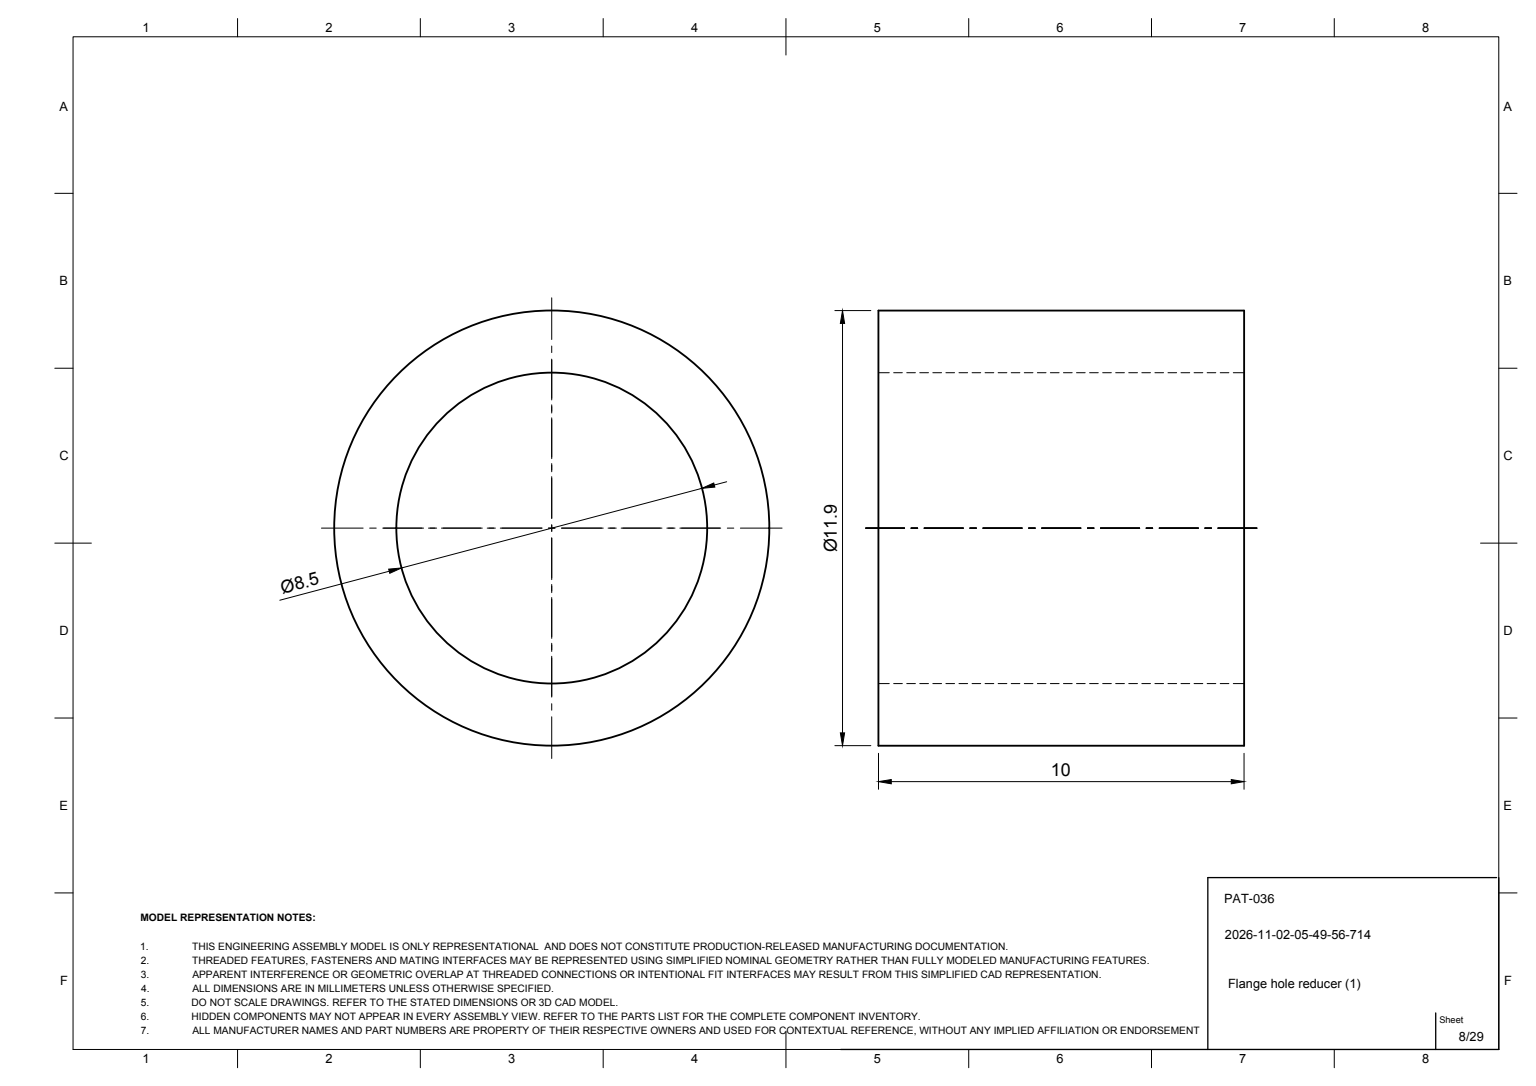
ISO-10303-21;
HEADER;
/* Generated by software containing ST-Developer
 * from STEP Tools, Inc. (www.steptools.com) 
 */

FILE_DESCRIPTION(
/* description */ ('Flange-mounted spindle'),
/* implementation_level */ '2;1');

FILE_NAME(
/* name */ 'Flange hole reducer (1).step',
/* time_stamp */ '2026-10-27T10:49:51-07:00',
/* author */ (''),
/* organization */ (''),
/* preprocessor_version */ 'ST-DEVELOPER v20.2',
/* originating_system */ 'Autodesk Translation Framework v15.17.0.0',
/* authorisation */ '');

FILE_SCHEMA (('AUTOMOTIVE_DESIGN { 1 0 10303 214 3 1 1 }'));
ENDSEC;

DATA;
#10=MECHANICAL_DESIGN_GEOMETRIC_PRESENTATION_REPRESENTATION('',(#341),#11764);
#287=SHAPE_REPRESENTATION_RELATIONSHIP('SRR','None',#11883,#314);
#314=ADVANCED_BREP_SHAPE_REPRESENTATION('',(#369),#11738);
#341=STYLED_ITEM('',(#12113),#369);
#369=MANIFOLD_SOLID_BREP('Body1',#6133);
#411=FACE_BOUND('',#1069,.T.);
#412=FACE_BOUND('',#1071,.T.);
#522=PLANE('',#6520);
#523=PLANE('',#6521);
#701=FACE_OUTER_BOUND('',#1066,.T.);
#702=FACE_OUTER_BOUND('',#1067,.T.);
#703=FACE_OUTER_BOUND('',#1068,.T.);
#704=FACE_OUTER_BOUND('',#1070,.T.);
#1066=EDGE_LOOP('',(#4131,#4132,#4133,#4134));
#1067=EDGE_LOOP('',(#4135,#4136,#4137,#4138));
#1068=EDGE_LOOP('',(#4139));
#1069=EDGE_LOOP('',(#4140));
#1070=EDGE_LOOP('',(#4141));
#1071=EDGE_LOOP('',(#4142));
#1520=LINE('',#9270,#1942);
#1521=LINE('',#9276,#1943);
#1942=VECTOR('',#7363,0.425);
#1943=VECTOR('',#7370,0.595);
#2345=CIRCLE('',#6515,0.425);
#2346=CIRCLE('',#6516,0.425);
#2347=CIRCLE('',#6518,0.595);
#2348=CIRCLE('',#6519,0.595);
#2691=VERTEX_POINT('',#9267);
#2692=VERTEX_POINT('',#9269);
#2693=VERTEX_POINT('',#9273);
#2694=VERTEX_POINT('',#9275);
#3258=EDGE_CURVE('',#2691,#2691,#2345,.T.);
#3259=EDGE_CURVE('',#2691,#2692,#1520,.T.);
#3260=EDGE_CURVE('',#2692,#2692,#2346,.T.);
#3261=EDGE_CURVE('',#2693,#2693,#2347,.T.);
#3262=EDGE_CURVE('',#2693,#2694,#1521,.T.);
#3263=EDGE_CURVE('',#2694,#2694,#2348,.T.);
#4131=ORIENTED_EDGE('',*,*,#3258,.F.);
#4132=ORIENTED_EDGE('',*,*,#3259,.T.);
#4133=ORIENTED_EDGE('',*,*,#3260,.T.);
#4134=ORIENTED_EDGE('',*,*,#3259,.F.);
#4135=ORIENTED_EDGE('',*,*,#3261,.F.);
#4136=ORIENTED_EDGE('',*,*,#3262,.T.);
#4137=ORIENTED_EDGE('',*,*,#3263,.T.);
#4138=ORIENTED_EDGE('',*,*,#3262,.F.);
#4139=ORIENTED_EDGE('',*,*,#3261,.T.);
#4140=ORIENTED_EDGE('',*,*,#3258,.T.);
#4141=ORIENTED_EDGE('',*,*,#3263,.F.);
#4142=ORIENTED_EDGE('',*,*,#3260,.F.);
#5636=CYLINDRICAL_SURFACE('',#6514,0.425);
#5637=CYLINDRICAL_SURFACE('',#6517,0.595);
#5812=ADVANCED_FACE('',(#701),#5636,.F.);
#5813=ADVANCED_FACE('',(#702),#5637,.T.);
#5814=ADVANCED_FACE('',(#703,#411),#522,.T.);
#5815=ADVANCED_FACE('',(#704,#412),#523,.F.);
#6133=CLOSED_SHELL('',(#5812,#5813,#5814,#5815));
#6513=AXIS2_PLACEMENT_3D('',#9265,#7357,#7358);
#6514=AXIS2_PLACEMENT_3D('',#9266,#7359,#7360);
#6515=AXIS2_PLACEMENT_3D('',#9268,#7361,#7362);
#6516=AXIS2_PLACEMENT_3D('',#9271,#7364,#7365);
#6517=AXIS2_PLACEMENT_3D('',#9272,#7366,#7367);
#6518=AXIS2_PLACEMENT_3D('',#9274,#7368,#7369);
#6519=AXIS2_PLACEMENT_3D('',#9277,#7371,#7372);
#6520=AXIS2_PLACEMENT_3D('',#9278,#7373,#7374);
#6521=AXIS2_PLACEMENT_3D('',#9279,#7375,#7376);
#7357=DIRECTION('axis',(0.,0.,1.));
#7358=DIRECTION('refdir',(1.,0.,0.));
#7359=DIRECTION('center_axis',(0.,1.,0.));
#7360=DIRECTION('ref_axis',(1.,0.,0.));
#7361=DIRECTION('center_axis',(0.,-1.,0.));
#7362=DIRECTION('ref_axis',(1.,0.,0.));
#7363=DIRECTION('',(0.,-1.,0.));
#7364=DIRECTION('center_axis',(0.,-1.,0.));
#7365=DIRECTION('ref_axis',(1.,0.,0.));
#7366=DIRECTION('center_axis',(0.,1.,0.));
#7367=DIRECTION('ref_axis',(1.,0.,0.));
#7368=DIRECTION('center_axis',(0.,1.,0.));
#7369=DIRECTION('ref_axis',(1.,0.,0.));
#7370=DIRECTION('',(0.,-1.,0.));
#7371=DIRECTION('center_axis',(0.,1.,0.));
#7372=DIRECTION('ref_axis',(1.,0.,0.));
#7373=DIRECTION('center_axis',(0.,1.,0.));
#7374=DIRECTION('ref_axis',(1.,0.,0.));
#7375=DIRECTION('center_axis',(0.,1.,0.));
#7376=DIRECTION('ref_axis',(1.,0.,0.));
#9265=CARTESIAN_POINT('',(0.,0.,0.));
#9266=CARTESIAN_POINT('Origin',(-3.2,-0.5,11.2));
#9267=CARTESIAN_POINT('',(-3.625,0.5,11.2));
#9268=CARTESIAN_POINT('Origin',(-3.2,0.5,11.2));
#9269=CARTESIAN_POINT('',(-3.625,-0.5,11.2));
#9270=CARTESIAN_POINT('',(-3.625,-0.5,11.2));
#9271=CARTESIAN_POINT('Origin',(-3.2,-0.5,11.2));
#9272=CARTESIAN_POINT('Origin',(-3.2,-0.5,11.2));
#9273=CARTESIAN_POINT('',(-3.795,0.5,11.2));
#9274=CARTESIAN_POINT('Origin',(-3.2,0.5,11.2));
#9275=CARTESIAN_POINT('',(-3.795,-0.5,11.2));
#9276=CARTESIAN_POINT('',(-3.795,-0.5,11.2));
#9277=CARTESIAN_POINT('Origin',(-3.2,-0.5,11.2));
#9278=CARTESIAN_POINT('Origin',(-3.2,0.5,11.2));
#9279=CARTESIAN_POINT('Origin',(-3.2,-0.5,11.2));
#11706=UNCERTAINTY_MEASURE_WITH_UNIT(LENGTH_MEASURE(0.001),#11765,
'DISTANCE_ACCURACY_VALUE',
'Maximum model space distance between geometric entities at asserted c
onnectivities');
#11732=UNCERTAINTY_MEASURE_WITH_UNIT(LENGTH_MEASURE(0.001),#11765,
'DISTANCE_ACCURACY_VALUE',
'Maximum model space distance between geometric entities at asserted c
onnectivities');
#11738=(
GEOMETRIC_REPRESENTATION_CONTEXT(3)
GLOBAL_UNCERTAINTY_ASSIGNED_CONTEXT((#11706))
GLOBAL_UNIT_ASSIGNED_CONTEXT((#11765,#11767,#11768))
REPRESENTATION_CONTEXT('','3D')
);
#11764=(
GEOMETRIC_REPRESENTATION_CONTEXT(3)
GLOBAL_UNCERTAINTY_ASSIGNED_CONTEXT((#11732))
GLOBAL_UNIT_ASSIGNED_CONTEXT((#11765,#11767,#11768))
REPRESENTATION_CONTEXT('','3D')
);
#11765=(
LENGTH_UNIT()
NAMED_UNIT(*)
SI_UNIT(.CENTI.,.METRE.)
);
#11767=(
NAMED_UNIT(*)
PLANE_ANGLE_UNIT()
SI_UNIT($,.RADIAN.)
);
#11768=(
NAMED_UNIT(*)
SI_UNIT($,.STERADIAN.)
SOLID_ANGLE_UNIT()
);
#11774=SHAPE_DEFINITION_REPRESENTATION(#11805,#11883);
#11805=PRODUCT_DEFINITION_SHAPE('',$,#11915);
#11883=SHAPE_REPRESENTATION('',(#6513),#11738);
#11909=PRODUCT_DEFINITION_CONTEXT('part definition',#12004,'design');
#11915=PRODUCT_DEFINITION('Flange hole reducer (1)',
'Flange hole reducer (1)',#11946,#11909);
#11946=PRODUCT_DEFINITION_FORMATION('',$,#12011);
#12004=APPLICATION_CONTEXT(
'Core Data for Automotive Mechanical Design Process');
#12005=PRODUCT_CONTEXT('part definition',#12004,'mechanical');
#12011=PRODUCT('Flange hole reducer (1)','Flange hole reducer (1)',
'Flange hole reducer (1)',(#12005));
#12107=COLOUR_RGB('Off White',0.89,0.88,0.83);
#12108=FILL_AREA_STYLE_COLOUR('',#12107);
#12109=FILL_AREA_STYLE('',(#12108));
#12110=SURFACE_STYLE_FILL_AREA(#12109);
#12111=SURFACE_SIDE_STYLE('',(#12110));
#12112=SURFACE_STYLE_USAGE(.BOTH.,#12111);
#12113=PRESENTATION_STYLE_ASSIGNMENT((#12112));
ENDSEC;
END-ISO-10303-21;
